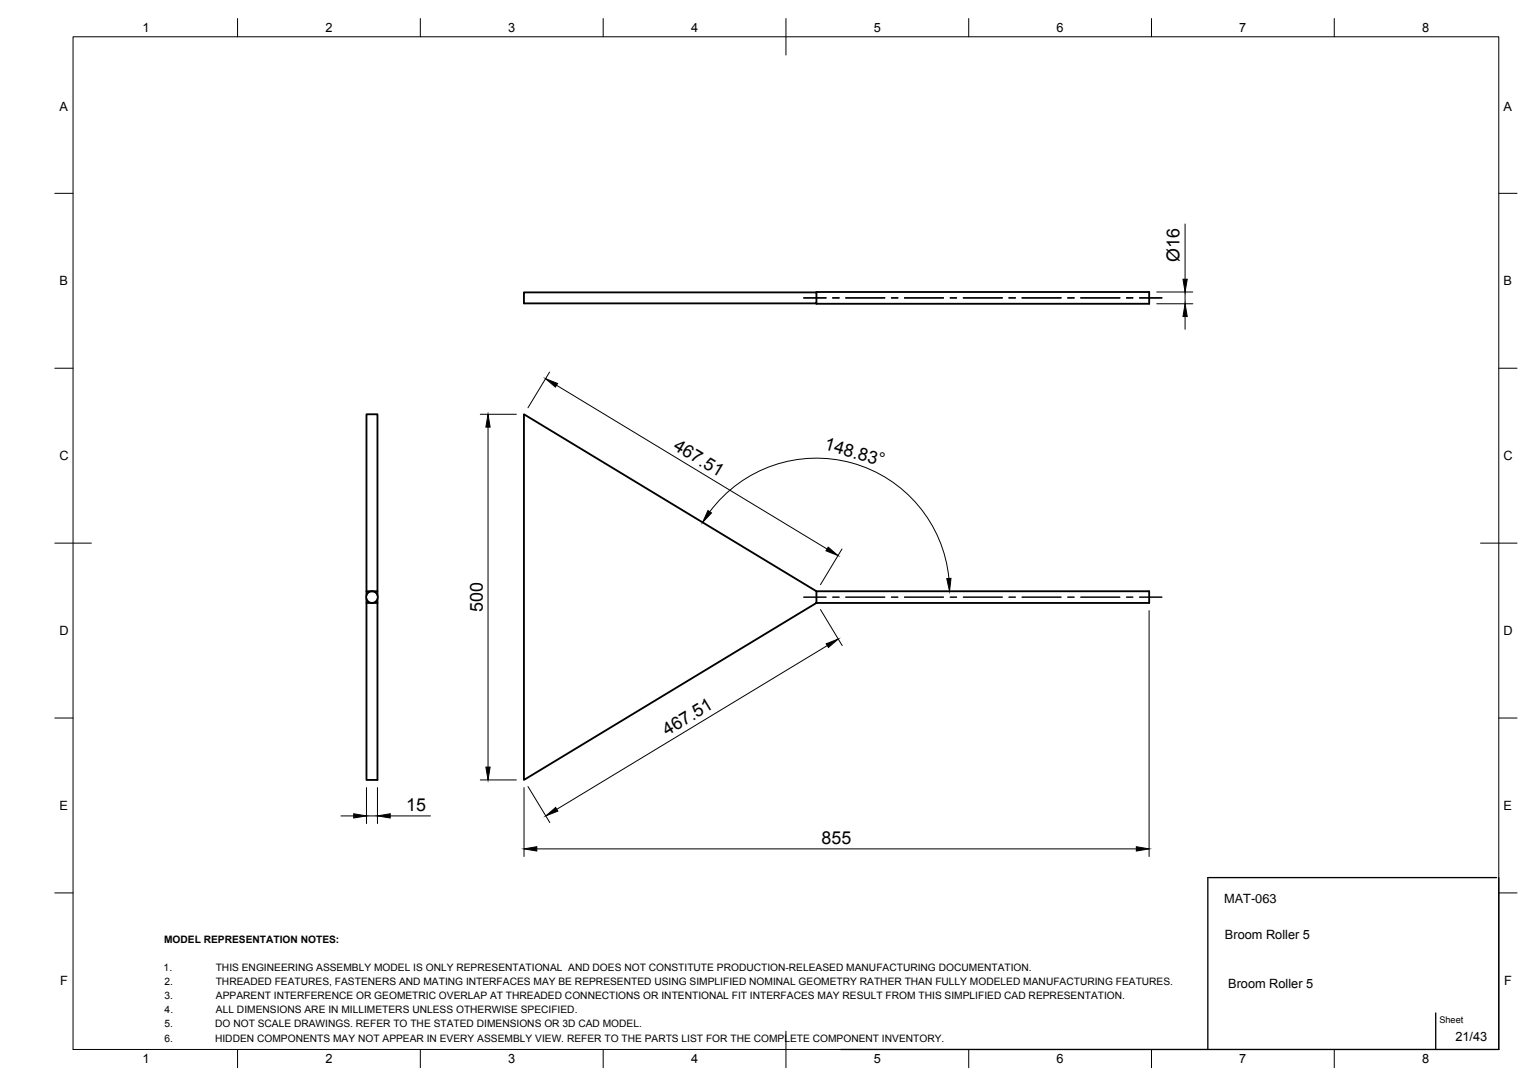
ISO-10303-21;
HEADER;
/* Generated by software containing ST-Developer
 * from STEP Tools, Inc. (www.steptools.com) 
 */

FILE_DESCRIPTION(
/* description */ (''),
/* implementation_level */ '2;1');

FILE_NAME(
/* name */ 'Broom Roller 5.step',
/* time_stamp */ '2026-10-24T09:43:01-07:00',
/* author */ (''),
/* organization */ (''),
/* preprocessor_version */ 'ST-DEVELOPER v20.2',
/* originating_system */ 'Autodesk Translation Framework v15.15.0.0',
/* authorisation */ '');

FILE_SCHEMA (('AUTOMOTIVE_DESIGN { 1 0 10303 214 3 1 1 }'));
ENDSEC;

DATA;
#10=MECHANICAL_DESIGN_GEOMETRIC_PRESENTATION_REPRESENTATION('',(#286),#11112);
#220=SHAPE_REPRESENTATION_RELATIONSHIP('SRR','None',#11244,#253);
#253=ADVANCED_BREP_SHAPE_REPRESENTATION('',(#319),#11089);
#286=STYLED_ITEM('',(#11426),#319);
#319=MANIFOLD_SOLID_BREP('Broom Roller 5',#6023);
#573=PLANE('',#6902);
#574=PLANE('',#6903);
#575=PLANE('',#6904);
#576=PLANE('',#6905);
#577=PLANE('',#6906);
#578=PLANE('',#6907);
#579=PLANE('',#6908);
#580=PLANE('',#6909);
#581=PLANE('',#6910);
#582=PLANE('',#6911);
#583=PLANE('',#6912);
#584=PLANE('',#6913);
#873=FACE_OUTER_BOUND('',#1312,.T.);
#874=FACE_OUTER_BOUND('',#1313,.T.);
#875=FACE_OUTER_BOUND('',#1314,.T.);
#876=FACE_OUTER_BOUND('',#1315,.T.);
#877=FACE_OUTER_BOUND('',#1316,.T.);
#878=FACE_OUTER_BOUND('',#1317,.T.);
#879=FACE_OUTER_BOUND('',#1318,.T.);
#880=FACE_OUTER_BOUND('',#1319,.T.);
#881=FACE_OUTER_BOUND('',#1320,.T.);
#882=FACE_OUTER_BOUND('',#1321,.T.);
#883=FACE_OUTER_BOUND('',#1322,.T.);
#884=FACE_OUTER_BOUND('',#1323,.T.);
#885=FACE_OUTER_BOUND('',#1324,.T.);
#1312=EDGE_LOOP('',(#4799,#4800,#4801,#4802,#4803,#4804,#4805,#4806,#4807,
#4808));
#1313=EDGE_LOOP('',(#4809));
#1314=EDGE_LOOP('',(#4810,#4811,#4812));
#1315=EDGE_LOOP('',(#4813,#4814,#4815));
#1316=EDGE_LOOP('',(#4816,#4817,#4818));
#1317=EDGE_LOOP('',(#4819,#4820));
#1318=EDGE_LOOP('',(#4821,#4822,#4823));
#1319=EDGE_LOOP('',(#4824,#4825,#4826));
#1320=EDGE_LOOP('',(#4827,#4828,#4829,#4830,#4831,#4832));
#1321=EDGE_LOOP('',(#4833,#4834,#4835,#4836,#4837));
#1322=EDGE_LOOP('',(#4838,#4839,#4840,#4841,#4842,#4843));
#1323=EDGE_LOOP('',(#4844,#4845,#4846,#4847,#4848));
#1324=EDGE_LOOP('',(#4849,#4850,#4851,#4852));
#1711=LINE('',#10241,#2070);
#1712=LINE('',#10250,#2071);
#1713=LINE('',#10253,#2072);
#1714=LINE('',#10254,#2073);
#1715=LINE('',#10257,#2074);
#1716=LINE('',#10258,#2075);
#1717=LINE('',#10260,#2076);
#1718=LINE('',#10263,#2077);
#1719=LINE('',#10264,#2078);
#1720=LINE('',#10267,#2079);
#1721=LINE('',#10268,#2080);
#1722=LINE('',#10271,#2081);
#1723=LINE('',#10273,#2082);
#1724=LINE('',#10274,#2083);
#1725=LINE('',#10277,#2084);
#1726=LINE('',#10278,#2085);
#1727=LINE('',#10281,#2086);
#1728=LINE('',#10282,#2087);
#1729=LINE('',#10284,#2088);
#2070=VECTOR('',#8395,0.0079999999576051);
#2071=VECTOR('',#8408,0.01);
#2072=VECTOR('',#8411,0.01);
#2073=VECTOR('',#8412,0.01);
#2074=VECTOR('',#8415,0.01);
#2075=VECTOR('',#8416,0.01);
#2076=VECTOR('',#8419,0.01);
#2077=VECTOR('',#8422,0.01);
#2078=VECTOR('',#8423,0.01);
#2079=VECTOR('',#8426,0.01);
#2080=VECTOR('',#8427,0.01);
#2081=VECTOR('',#8430,0.01);
#2082=VECTOR('',#8431,0.01);
#2083=VECTOR('',#8432,0.01);
#2084=VECTOR('',#8435,0.01);
#2085=VECTOR('',#8436,0.01);
#2086=VECTOR('',#8439,0.01);
#2087=VECTOR('',#8440,0.01);
#2088=VECTOR('',#8443,0.01);
#2546=CIRCLE('',#6894,0.0079999999576051);
#2547=CIRCLE('',#6895,0.0079999999576051);
#2548=CIRCLE('',#6896,0.0079999999576051);
#2549=CIRCLE('',#6897,0.0079999999576051);
#2550=CIRCLE('',#6898,0.0079999999576051);
#2551=CIRCLE('',#6899,0.0079999999576051);
#2552=CIRCLE('',#6900,0.0079999999576051);
#2553=CIRCLE('',#6901,0.0079999999576051);
#2948=VERTEX_POINT('',#10231);
#2949=VERTEX_POINT('',#10232);
#2950=VERTEX_POINT('',#10234);
#2951=VERTEX_POINT('',#10236);
#2952=VERTEX_POINT('',#10238);
#2953=VERTEX_POINT('',#10240);
#2954=VERTEX_POINT('',#10243);
#2955=VERTEX_POINT('',#10245);
#2956=VERTEX_POINT('',#10252);
#2957=VERTEX_POINT('',#10256);
#2958=VERTEX_POINT('',#10262);
#2959=VERTEX_POINT('',#10266);
#2960=VERTEX_POINT('',#10270);
#2961=VERTEX_POINT('',#10272);
#2962=VERTEX_POINT('',#10276);
#2963=VERTEX_POINT('',#10280);
#3603=EDGE_CURVE('',#2948,#2949,#2546,.F.);
#3604=EDGE_CURVE('',#2949,#2950,#2547,.F.);
#3605=EDGE_CURVE('',#2950,#2951,#2548,.F.);
#3606=EDGE_CURVE('',#2951,#2952,#2549,.F.);
#3607=EDGE_CURVE('',#2952,#2953,#1711,.T.);
#3608=EDGE_CURVE('',#2953,#2953,#2550,.T.);
#3609=EDGE_CURVE('',#2952,#2954,#2551,.F.);
#3610=EDGE_CURVE('',#2954,#2955,#2552,.F.);
#3611=EDGE_CURVE('',#2955,#2948,#2553,.F.);
#3612=EDGE_CURVE('',#2951,#2954,#1712,.T.);
#3613=EDGE_CURVE('',#2956,#2955,#1713,.T.);
#3614=EDGE_CURVE('',#2954,#2956,#1714,.T.);
#3615=EDGE_CURVE('',#2957,#2948,#1715,.T.);
#3616=EDGE_CURVE('',#2955,#2957,#1716,.T.);
#3617=EDGE_CURVE('',#2948,#2949,#1717,.T.);
#3618=EDGE_CURVE('',#2958,#2950,#1718,.T.);
#3619=EDGE_CURVE('',#2949,#2958,#1719,.T.);
#3620=EDGE_CURVE('',#2959,#2951,#1720,.T.);
#3621=EDGE_CURVE('',#2950,#2959,#1721,.T.);
#3622=EDGE_CURVE('',#2960,#2959,#1722,.T.);
#3623=EDGE_CURVE('',#2961,#2960,#1723,.T.);
#3624=EDGE_CURVE('',#2956,#2961,#1724,.T.);
#3625=EDGE_CURVE('',#2962,#2961,#1725,.T.);
#3626=EDGE_CURVE('',#2957,#2962,#1726,.T.);
#3627=EDGE_CURVE('',#2962,#2963,#1727,.T.);
#3628=EDGE_CURVE('',#2963,#2958,#1728,.T.);
#3629=EDGE_CURVE('',#2963,#2960,#1729,.T.);
#4799=ORIENTED_EDGE('',*,*,#3603,.T.);
#4800=ORIENTED_EDGE('',*,*,#3604,.T.);
#4801=ORIENTED_EDGE('',*,*,#3605,.T.);
#4802=ORIENTED_EDGE('',*,*,#3606,.T.);
#4803=ORIENTED_EDGE('',*,*,#3607,.T.);
#4804=ORIENTED_EDGE('',*,*,#3608,.T.);
#4805=ORIENTED_EDGE('',*,*,#3607,.F.);
#4806=ORIENTED_EDGE('',*,*,#3609,.T.);
#4807=ORIENTED_EDGE('',*,*,#3610,.T.);
#4808=ORIENTED_EDGE('',*,*,#3611,.T.);
#4809=ORIENTED_EDGE('',*,*,#3608,.F.);
#4810=ORIENTED_EDGE('',*,*,#3612,.T.);
#4811=ORIENTED_EDGE('',*,*,#3609,.F.);
#4812=ORIENTED_EDGE('',*,*,#3606,.F.);
#4813=ORIENTED_EDGE('',*,*,#3613,.T.);
#4814=ORIENTED_EDGE('',*,*,#3610,.F.);
#4815=ORIENTED_EDGE('',*,*,#3614,.T.);
#4816=ORIENTED_EDGE('',*,*,#3615,.T.);
#4817=ORIENTED_EDGE('',*,*,#3611,.F.);
#4818=ORIENTED_EDGE('',*,*,#3616,.T.);
#4819=ORIENTED_EDGE('',*,*,#3617,.T.);
#4820=ORIENTED_EDGE('',*,*,#3603,.F.);
#4821=ORIENTED_EDGE('',*,*,#3618,.T.);
#4822=ORIENTED_EDGE('',*,*,#3604,.F.);
#4823=ORIENTED_EDGE('',*,*,#3619,.T.);
#4824=ORIENTED_EDGE('',*,*,#3620,.T.);
#4825=ORIENTED_EDGE('',*,*,#3605,.F.);
#4826=ORIENTED_EDGE('',*,*,#3621,.T.);
#4827=ORIENTED_EDGE('',*,*,#3622,.F.);
#4828=ORIENTED_EDGE('',*,*,#3623,.F.);
#4829=ORIENTED_EDGE('',*,*,#3624,.F.);
#4830=ORIENTED_EDGE('',*,*,#3614,.F.);
#4831=ORIENTED_EDGE('',*,*,#3612,.F.);
#4832=ORIENTED_EDGE('',*,*,#3620,.F.);
#4833=ORIENTED_EDGE('',*,*,#3613,.F.);
#4834=ORIENTED_EDGE('',*,*,#3624,.T.);
#4835=ORIENTED_EDGE('',*,*,#3625,.F.);
#4836=ORIENTED_EDGE('',*,*,#3626,.F.);
#4837=ORIENTED_EDGE('',*,*,#3616,.F.);
#4838=ORIENTED_EDGE('',*,*,#3627,.T.);
#4839=ORIENTED_EDGE('',*,*,#3628,.T.);
#4840=ORIENTED_EDGE('',*,*,#3619,.F.);
#4841=ORIENTED_EDGE('',*,*,#3617,.F.);
#4842=ORIENTED_EDGE('',*,*,#3615,.F.);
#4843=ORIENTED_EDGE('',*,*,#3626,.T.);
#4844=ORIENTED_EDGE('',*,*,#3622,.T.);
#4845=ORIENTED_EDGE('',*,*,#3621,.F.);
#4846=ORIENTED_EDGE('',*,*,#3618,.F.);
#4847=ORIENTED_EDGE('',*,*,#3628,.F.);
#4848=ORIENTED_EDGE('',*,*,#3629,.T.);
#4849=ORIENTED_EDGE('',*,*,#3625,.T.);
#4850=ORIENTED_EDGE('',*,*,#3623,.T.);
#4851=ORIENTED_EDGE('',*,*,#3629,.F.);
#4852=ORIENTED_EDGE('',*,*,#3627,.F.);
#5574=CYLINDRICAL_SURFACE('',#6893,0.0079999999576051);
#5846=ADVANCED_FACE('',(#873),#5574,.T.);
#5847=ADVANCED_FACE('',(#874),#573,.F.);
#5848=ADVANCED_FACE('',(#875),#574,.T.);
#5849=ADVANCED_FACE('',(#876),#575,.T.);
#5850=ADVANCED_FACE('',(#877),#576,.T.);
#5851=ADVANCED_FACE('',(#878),#577,.T.);
#5852=ADVANCED_FACE('',(#879),#578,.T.);
#5853=ADVANCED_FACE('',(#880),#579,.T.);
#5854=ADVANCED_FACE('',(#881),#580,.F.);
#5855=ADVANCED_FACE('',(#882),#581,.F.);
#5856=ADVANCED_FACE('',(#883),#582,.T.);
#5857=ADVANCED_FACE('',(#884),#583,.T.);
#5858=ADVANCED_FACE('',(#885),#584,.F.);
#6023=CLOSED_SHELL('',(#5846,#5847,#5848,#5849,#5850,#5851,#5852,#5853,
#5854,#5855,#5856,#5857,#5858));
#6892=AXIS2_PLACEMENT_3D('',#10229,#8383,#8384);
#6893=AXIS2_PLACEMENT_3D('',#10230,#8385,#8386);
#6894=AXIS2_PLACEMENT_3D('',#10233,#8387,#8388);
#6895=AXIS2_PLACEMENT_3D('',#10235,#8389,#8390);
#6896=AXIS2_PLACEMENT_3D('',#10237,#8391,#8392);
#6897=AXIS2_PLACEMENT_3D('',#10239,#8393,#8394);
#6898=AXIS2_PLACEMENT_3D('',#10242,#8396,#8397);
#6899=AXIS2_PLACEMENT_3D('',#10244,#8398,#8399);
#6900=AXIS2_PLACEMENT_3D('',#10246,#8400,#8401);
#6901=AXIS2_PLACEMENT_3D('',#10247,#8402,#8403);
#6902=AXIS2_PLACEMENT_3D('',#10248,#8404,#8405);
#6903=AXIS2_PLACEMENT_3D('',#10249,#8406,#8407);
#6904=AXIS2_PLACEMENT_3D('',#10251,#8409,#8410);
#6905=AXIS2_PLACEMENT_3D('',#10255,#8413,#8414);
#6906=AXIS2_PLACEMENT_3D('',#10259,#8417,#8418);
#6907=AXIS2_PLACEMENT_3D('',#10261,#8420,#8421);
#6908=AXIS2_PLACEMENT_3D('',#10265,#8424,#8425);
#6909=AXIS2_PLACEMENT_3D('',#10269,#8428,#8429);
#6910=AXIS2_PLACEMENT_3D('',#10275,#8433,#8434);
#6911=AXIS2_PLACEMENT_3D('',#10279,#8437,#8438);
#6912=AXIS2_PLACEMENT_3D('',#10283,#8441,#8442);
#6913=AXIS2_PLACEMENT_3D('',#10285,#8444,#8445);
#8383=DIRECTION('axis',(0.,0.,1.));
#8384=DIRECTION('refdir',(1.,0.,0.));
#8385=DIRECTION('center_axis',(0.,0.388095893919631,-0.92161899780914));
#8386=DIRECTION('ref_axis',(0.,0.921618997809139,0.388095893919631));
#8387=DIRECTION('center_axis',(0.,0.388095893919631,-0.92161899780914));
#8388=DIRECTION('ref_axis',(0.,0.921618997809139,0.388095893919631));
#8389=DIRECTION('center_axis',(0.,0.388095893919631,-0.92161899780914));
#8390=DIRECTION('ref_axis',(0.,0.921618997809139,0.388095893919631));
#8391=DIRECTION('center_axis',(0.,0.388095893919631,-0.92161899780914));
#8392=DIRECTION('ref_axis',(0.,0.921618997809139,0.388095893919631));
#8393=DIRECTION('center_axis',(0.,0.388095893919631,-0.92161899780914));
#8394=DIRECTION('ref_axis',(0.,0.921618997809139,0.388095893919631));
#8395=DIRECTION('',(0.,-0.388095893919631,0.921618997809139));
#8396=DIRECTION('center_axis',(0.,0.388095893919631,-0.92161899780914));
#8397=DIRECTION('ref_axis',(0.,0.921618997809139,0.388095893919631));
#8398=DIRECTION('center_axis',(0.,0.388095893919631,-0.92161899780914));
#8399=DIRECTION('ref_axis',(0.,0.921618997809139,0.388095893919631));
#8400=DIRECTION('center_axis',(0.,0.388095893919631,-0.92161899780914));
#8401=DIRECTION('ref_axis',(0.,0.921618997809139,0.388095893919631));
#8402=DIRECTION('center_axis',(0.,0.388095893919631,-0.92161899780914));
#8403=DIRECTION('ref_axis',(0.,0.921618997809139,0.388095893919631));
#8404=DIRECTION('center_axis',(1.75398457025153E-15,0.388095852305965,-0.921619015332749));
#8405=DIRECTION('ref_axis',(3.06157850855551E-32,0.921619015332749,0.388095852305965));
#8406=DIRECTION('center_axis',(2.26659755541862E-15,0.388095750770971,-0.921619058089359));
#8407=DIRECTION('ref_axis',(3.64804420840904E-32,0.921619058089359,0.388095750770971));
#8408=DIRECTION('',(1.,0.,0.));
#8409=DIRECTION('center_axis',(2.22848289163665E-15,-0.388095804062443,
0.921619035648204));
#8410=DIRECTION('ref_axis',(-1.35081649158113E-31,-0.921619035648204,-0.388095804062443));
#8411=DIRECTION('',(4.2446461003979E-8,0.921619025681862,0.388095827729717));
#8412=DIRECTION('',(1.,0.,0.));
#8413=DIRECTION('center_axis',(-1.49720831504864E-15,-0.388095851468213,
0.921619015685529));
#8414=DIRECTION('ref_axis',(-1.5492957769102E-32,-0.921619015685529,-0.388095851468213));
#8415=DIRECTION('',(-1.,0.,0.));
#8416=DIRECTION('',(1.96652829206634E-8,0.921619011068175,0.388095862433136));
#8417=DIRECTION('center_axis',(-8.05371050902293E-15,0.388095039684462,
-0.921619357529081));
#8418=DIRECTION('ref_axis',(-4.42778246385967E-33,0.921619357529081,0.388095039684462));
#8419=DIRECTION('',(-1.,0.,0.));
#8420=DIRECTION('center_axis',(-1.48913479951885E-15,-0.388095851468213,
0.921619015685529));
#8421=DIRECTION('ref_axis',(3.33947309911167E-32,-0.921619015685529,-0.388095851468213));
#8422=DIRECTION('',(1.96652829206634E-8,-0.921619011068175,-0.388095862433136));
#8423=DIRECTION('',(-1.,0.,0.));
#8424=DIRECTION('center_axis',(2.25639593240362E-15,-0.388095804062443,
0.921619035648204));
#8425=DIRECTION('ref_axis',(-1.14895763187271E-31,-0.921619035648204,-0.388095804062443));
#8426=DIRECTION('',(1.,0.,0.));
#8427=DIRECTION('',(4.2446461003979E-8,-0.921619025681862,-0.388095827729717));
#8428=DIRECTION('center_axis',(4.13124616662422E-17,0.921618997376154,0.388095894947849));
#8429=DIRECTION('ref_axis',(-4.90455258387228E-34,-0.388095894947849,0.921618997376154));
#8430=DIRECTION('',(0.517637880705175,-0.332054771617521,0.788537033439198));
#8431=DIRECTION('',(-1.,0.,0.));
#8432=DIRECTION('',(0.517637880705175,0.332054771617521,-0.788537033439198));
#8433=DIRECTION('center_axis',(-0.855599803914806,0.200893135247141,-0.477064905176978));
#8434=DIRECTION('ref_axis',(-0.486993155484724,-9.98976039519683E-17,0.873405785709616));
#8435=DIRECTION('',(-6.49786640054161E-9,-0.921618997845643,-0.388095893832946));
#8436=DIRECTION('',(0.517637880705176,0.332054769800693,-0.788537034204268));
#8437=DIRECTION('center_axis',(-1.84726342759314E-17,0.921618998270346,
0.388095892824394));
#8438=DIRECTION('ref_axis',(3.04412378032587E-35,-0.388095892824394,0.921618998270346));
#8439=DIRECTION('',(-1.,0.,0.));
#8440=DIRECTION('',(0.517637880705175,-0.332054769800693,0.788537034204268));
#8441=DIRECTION('center_axis',(-0.855599803914806,-0.200893135247141,0.477064905176978));
#8442=DIRECTION('ref_axis',(0.486993155484724,-9.98976039519683E-17,0.873405785709616));
#8443=DIRECTION('',(6.49786640054161E-9,-0.921618997845643,-0.388095893832946));
#8444=DIRECTION('center_axis',(8.66968723023857E-18,-0.388095893832947,
0.921618997845642));
#8445=DIRECTION('ref_axis',(-1.74143232952537E-34,-0.921618997845642,-0.388095893832947));
#10229=CARTESIAN_POINT('',(0.,0.,0.));
#10230=CARTESIAN_POINT('Origin',(0.,0.367464315,1.058527145));
#10231=CARTESIAN_POINT('',(0.00278388280878993,0.550960089028251,0.64210121993291));
#10232=CARTESIAN_POINT('',(-0.00278388280878729,0.550960089028251,0.64210121993291));
#10233=CARTESIAN_POINT('Origin',(0.,0.544047946829229,0.63919050076935));
#10234=CARTESIAN_POINT('',(-0.00800000011528736,0.544047946993585,0.639190501008153));
#10235=CARTESIAN_POINT('Origin',(0.,0.544047946829229,0.63919050076935));
#10236=CARTESIAN_POINT('',(-0.00278388196528325,0.537135804154995,0.636279781774966));
#10237=CARTESIAN_POINT('Origin',(0.,0.544047946829229,0.63919050076935));
#10238=CARTESIAN_POINT('',(-9.79717434126005E-19,0.536674994885828,0.636085733634446));
#10239=CARTESIAN_POINT('Origin',(0.,0.544047946829229,0.63919050076935));
#10240=CARTESIAN_POINT('',(-9.79717434126005E-19,0.360091363113376,1.05542237773027));
#10241=CARTESIAN_POINT('',(-9.79717434126005E-19,0.360091363056599,1.0554223778651));
#10242=CARTESIAN_POINT('Origin',(0.,0.367464315056776,1.05852714486517));
#10243=CARTESIAN_POINT('',(0.00278388196528327,0.537135804154995,0.636279781774966));
#10244=CARTESIAN_POINT('Origin',(0.,0.544047946829229,0.63919050076935));
#10245=CARTESIAN_POINT('',(0.00800000011528736,0.544047946993585,0.639190501008153));
#10246=CARTESIAN_POINT('Origin',(0.,0.544047946829229,0.63919050076935));
#10247=CARTESIAN_POINT('Origin',(0.,0.544047946829229,0.63919050076935));
#10248=CARTESIAN_POINT('Origin',(-1.99493199737333E-19,0.3674643155,1.058527145));
#10249=CARTESIAN_POINT('Origin',(-2.16840434497101E-21,0.536905399427502,
0.636182758143169));
#10250=CARTESIAN_POINT('',(-0.00278388206046941,0.537135804,0.636279782));
#10251=CARTESIAN_POINT('Origin',(0.0053919408556245,0.540591875569578,0.637735141343516));
#10252=CARTESIAN_POINT('',(0.00800000011643423,0.537135803986997,0.636279782030879));
#10253=CARTESIAN_POINT('',(0.00800000010679859,0.537135803974924,0.636279782059549));
#10254=CARTESIAN_POINT('',(0.00278388206046941,0.537135804,0.636279782));
#10255=CARTESIAN_POINT('Origin',(0.0053919408556245,0.54750401792744,0.640645860656483));
#10256=CARTESIAN_POINT('',(0.00800000029334438,0.550960088967523,0.642101220077123));
#10257=CARTESIAN_POINT('',(0.00800000000000001,0.550960089,0.642101219999999));
#10258=CARTESIAN_POINT('',(0.0080000001207922,0.544047946835306,0.639190501384019));
#10259=CARTESIAN_POINT('Origin',(-2.16840434497101E-21,0.551190494069516,
0.642198243856831));
#10260=CARTESIAN_POINT('',(0.00278388206047068,0.550960089,0.64210122));
#10261=CARTESIAN_POINT('Origin',(-0.00539194085562444,0.54750401792744,
0.640645860656483));
#10262=CARTESIAN_POINT('',(-0.00800000029336689,0.550960088967528,0.642101220077111));
#10263=CARTESIAN_POINT('',(-0.00800000026828181,0.550960088937008,0.642101220149587));
#10264=CARTESIAN_POINT('',(-0.00278388206047068,0.550960089,0.642101219999999));
#10265=CARTESIAN_POINT('Origin',(-0.00539194085562444,0.540591875569578,
0.637735141343516));
#10266=CARTESIAN_POINT('',(-0.00800000011643421,0.537135803986997,0.636279782030879));
#10267=CARTESIAN_POINT('',(-0.00799999999999999,0.537135804,0.636279782));
#10268=CARTESIAN_POINT('',(-0.00800000042514707,0.544047947030544,0.639190500920384));
#10269=CARTESIAN_POINT('Origin',(-8.88178419700125E-18,0.614754983000001,
0.4519559825));
#10270=CARTESIAN_POINT('',(-0.249999999824503,0.69237416199696,0.267632183007222));
#10271=CARTESIAN_POINT('',(-0.249999999805892,0.692374161959955,0.267632183095097));
#10272=CARTESIAN_POINT('',(0.249999999824503,0.69237416199696,0.267632183007222));
#10273=CARTESIAN_POINT('',(0.249999999800628,0.692374162000001,0.267632183));
#10274=CARTESIAN_POINT('',(0.0080000001300884,0.537135803989865,0.636279782024071));
#10275=CARTESIAN_POINT('Origin',(0.129,0.621667125,0.4548667015));
#10276=CARTESIAN_POINT('',(0.249999999874932,0.706198446001423,0.273453620996678));
#10277=CARTESIAN_POINT('',(0.249999999890418,0.706198446007047,0.273453621002968));
#10278=CARTESIAN_POINT('',(0.00800000026828148,0.550960088937008,0.642101220149588));
#10279=CARTESIAN_POINT('Origin',(-8.88178419700125E-18,0.6285792675,0.457777420499999));
#10280=CARTESIAN_POINT('',(-0.249999999874803,0.706198446001377,0.273453620996738));
#10281=CARTESIAN_POINT('',(0.249999999800628,0.706198446,0.273453621));
#10282=CARTESIAN_POINT('',(-0.249999999795491,0.706198445962397,0.273453621089297));
#10283=CARTESIAN_POINT('Origin',(-0.129,0.621667125,0.4548667015));
#10284=CARTESIAN_POINT('',(-0.249999999890418,0.706198446007047,0.273453621002968));
#10285=CARTESIAN_POINT('Origin',(-8.88178419700125E-18,0.699286304,0.270542902));
#11050=UNCERTAINTY_MEASURE_WITH_UNIT(LENGTH_MEASURE(1.E-5),#11113,
'DISTANCE_ACCURACY_VALUE',
'Maximum model space distance between geometric entities at asserted c
onnectivities');
#11073=UNCERTAINTY_MEASURE_WITH_UNIT(LENGTH_MEASURE(1.E-5),#11113,
'DISTANCE_ACCURACY_VALUE',
'Maximum model space distance between geometric entities at asserted c
onnectivities');
#11089=(
GEOMETRIC_REPRESENTATION_CONTEXT(3)
GLOBAL_UNCERTAINTY_ASSIGNED_CONTEXT((#11050))
GLOBAL_UNIT_ASSIGNED_CONTEXT((#11113,#11114,#11115))
REPRESENTATION_CONTEXT('','3D')
);
#11112=(
GEOMETRIC_REPRESENTATION_CONTEXT(3)
GLOBAL_UNCERTAINTY_ASSIGNED_CONTEXT((#11073))
GLOBAL_UNIT_ASSIGNED_CONTEXT((#11113,#11114,#11115))
REPRESENTATION_CONTEXT('','3D')
);
#11113=(
LENGTH_UNIT()
NAMED_UNIT(*)
SI_UNIT($,.METRE.)
);
#11114=(
NAMED_UNIT(*)
PLANE_ANGLE_UNIT()
SI_UNIT($,.RADIAN.)
);
#11115=(
NAMED_UNIT(*)
SI_UNIT($,.STERADIAN.)
SOLID_ANGLE_UNIT()
);
#11131=SHAPE_DEFINITION_REPRESENTATION(#11169,#11244);
#11169=PRODUCT_DEFINITION_SHAPE('',$,#11283);
#11244=SHAPE_REPRESENTATION('',(#6892),#11089);
#11267=PRODUCT_DEFINITION_CONTEXT('part definition',#11383,'design');
#11283=PRODUCT_DEFINITION('Broom Roller 5','Broom Roller 5',#11321,#11267);
#11321=PRODUCT_DEFINITION_FORMATION('',$,#11400);
#11383=APPLICATION_CONTEXT(
'Core Data for Automotive Mechanical Design Process');
#11384=PRODUCT_CONTEXT('part definition',#11383,'mechanical');
#11400=PRODUCT('Broom Roller 5','Broom Roller 5',
'broom_and_roller__ DE     6575',(#11384));
#11426=PRESENTATION_STYLE_ASSIGNMENT((#11430));
#11430=SURFACE_STYLE_USAGE(.BOTH.,#11434);
#11434=SURFACE_SIDE_STYLE('',(#11438));
#11438=SURFACE_STYLE_FILL_AREA(#11442);
#11442=FILL_AREA_STYLE('Opaque(202,209,238)',(#11446));
#11446=FILL_AREA_STYLE_COLOUR('Opaque(202,209,238)',#11450);
#11450=COLOUR_RGB('Opaque(202,209,238)',0.792156862745098,0.819607843137255,
0.933333333333333);
ENDSEC;
END-ISO-10303-21;
